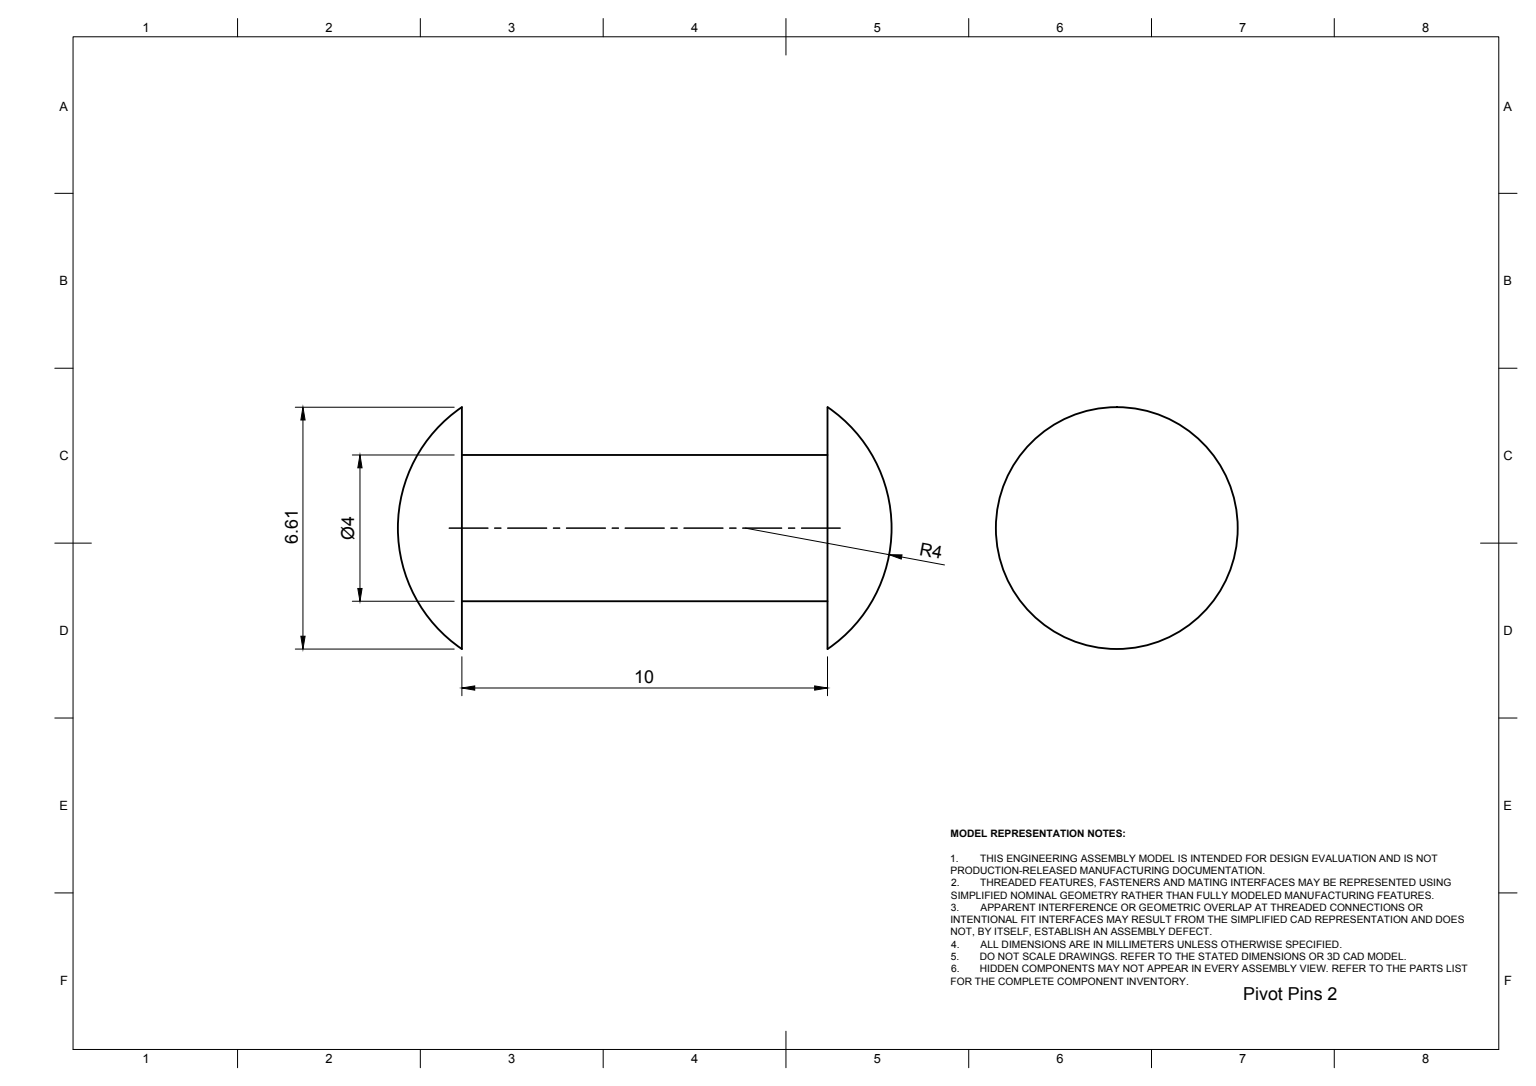
ISO-10303-21;
HEADER;
/* Generated by software containing ST-Developer
 * from STEP Tools, Inc. (www.steptools.com) 
 */

FILE_DESCRIPTION(
/* description */ ('STEP AP214'),
/* implementation_level */ '2;1');

FILE_NAME(
/* name */ 'Pivot Pins 2.step',
/* time_stamp */ '2026-10-06T11:11:25-07:00',
/* author */ (''),
/* organization */ (''),
/* preprocessor_version */ 'ST-DEVELOPER v20.2',
/* originating_system */ 'Autodesk Translation Framework v15.15.0.0',
/* authorisation */ '');

FILE_SCHEMA (('AUTOMOTIVE_DESIGN { 1 0 10303 214 3 1 1 }'));
ENDSEC;

DATA;
#10=MECHANICAL_DESIGN_GEOMETRIC_PRESENTATION_REPRESENTATION('',(#707),#47717);
#683=SHAPE_REPRESENTATION_RELATIONSHIP('SRR','None',#47770,#695);
#695=ADVANCED_BREP_SHAPE_REPRESENTATION('',(#719),#47714);
#707=STYLED_ITEM('',(#47830),#719);
#719=MANIFOLD_SOLID_BREP('Body1',#8934);
#751=FACE_BOUND('',#3058,.T.);
#752=FACE_BOUND('',#3060,.T.);
#871=PLANE('',#9832);
#872=PLANE('',#9833);
#1330=LINE('',#45925,#1817);
#1817=VECTOR('',#11921,2.);
#2041=CYLINDRICAL_SURFACE('',#9827,2.);
#2513=FACE_OUTER_BOUND('',#3054,.T.);
#2514=FACE_OUTER_BOUND('',#3055,.T.);
#2515=FACE_OUTER_BOUND('',#3056,.T.);
#2516=FACE_OUTER_BOUND('',#3057,.T.);
#2517=FACE_OUTER_BOUND('',#3059,.T.);
#3054=EDGE_LOOP('',(#8115));
#3055=EDGE_LOOP('',(#8116,#8117,#8118,#8119));
#3056=EDGE_LOOP('',(#8120));
#3057=EDGE_LOOP('',(#8121));
#3058=EDGE_LOOP('',(#8122));
#3059=EDGE_LOOP('',(#8123));
#3060=EDGE_LOOP('',(#8124));
#3468=CIRCLE('',#9826,3.30718913883074);
#3469=CIRCLE('',#9828,2.);
#3470=CIRCLE('',#9829,2.);
#3471=CIRCLE('',#9831,3.30718913883074);
#4301=VERTEX_POINT('',#45919);
#4302=VERTEX_POINT('',#45922);
#4303=VERTEX_POINT('',#45924);
#4304=VERTEX_POINT('',#45928);
#5583=EDGE_CURVE('',#4301,#4301,#3468,.T.);
#5584=EDGE_CURVE('',#4302,#4302,#3469,.T.);
#5585=EDGE_CURVE('',#4302,#4303,#1330,.T.);
#5586=EDGE_CURVE('',#4303,#4303,#3470,.T.);
#5587=EDGE_CURVE('',#4304,#4304,#3471,.T.);
#8115=ORIENTED_EDGE('',*,*,#5583,.T.);
#8116=ORIENTED_EDGE('',*,*,#5584,.F.);
#8117=ORIENTED_EDGE('',*,*,#5585,.T.);
#8118=ORIENTED_EDGE('',*,*,#5586,.T.);
#8119=ORIENTED_EDGE('',*,*,#5585,.F.);
#8120=ORIENTED_EDGE('',*,*,#5587,.F.);
#8121=ORIENTED_EDGE('',*,*,#5587,.T.);
#8122=ORIENTED_EDGE('',*,*,#5586,.F.);
#8123=ORIENTED_EDGE('',*,*,#5583,.F.);
#8124=ORIENTED_EDGE('',*,*,#5584,.T.);
#8411=SPHERICAL_SURFACE('',#9825,4.);
#8412=SPHERICAL_SURFACE('',#9830,4.);
#8863=ADVANCED_FACE('',(#2513),#8411,.T.);
#8864=ADVANCED_FACE('',(#2514),#2041,.T.);
#8865=ADVANCED_FACE('',(#2515),#8412,.T.);
#8866=ADVANCED_FACE('',(#2516,#751),#871,.T.);
#8867=ADVANCED_FACE('',(#2517,#752),#872,.T.);
#8934=CLOSED_SHELL('',(#8863,#8864,#8865,#8866,#8867));
#9824=AXIS2_PLACEMENT_3D('',#45917,#11911,#11912);
#9825=AXIS2_PLACEMENT_3D('',#45918,#11913,#11914);
#9826=AXIS2_PLACEMENT_3D('',#45920,#11915,#11916);
#9827=AXIS2_PLACEMENT_3D('',#45921,#11917,#11918);
#9828=AXIS2_PLACEMENT_3D('',#45923,#11919,#11920);
#9829=AXIS2_PLACEMENT_3D('',#45926,#11922,#11923);
#9830=AXIS2_PLACEMENT_3D('',#45927,#11924,#11925);
#9831=AXIS2_PLACEMENT_3D('',#45929,#11926,#11927);
#9832=AXIS2_PLACEMENT_3D('',#45930,#11928,#11929);
#9833=AXIS2_PLACEMENT_3D('',#45931,#11930,#11931);
#11911=DIRECTION('axis',(0.,0.,1.));
#11912=DIRECTION('refdir',(1.,0.,0.));
#11913=DIRECTION('center_axis',(0.00483401456277122,-0.999988316083346,
0.));
#11914=DIRECTION('ref_axis',(0.999988316083346,0.00483401456277122,0.));
#11915=DIRECTION('center_axis',(2.50063434304146E-17,1.27632226958495E-16,
1.));
#11916=DIRECTION('ref_axis',(0.00483401456277147,-0.999988316083347,1.27509854685889E-16));
#11917=DIRECTION('center_axis',(2.50063434304146E-17,1.27632226958495E-16,
1.));
#11918=DIRECTION('ref_axis',(0.00483401456276983,-0.999988316083346,1.27509854685889E-16));
#11919=DIRECTION('center_axis',(2.50063434304146E-17,1.27632226958495E-16,
1.));
#11920=DIRECTION('ref_axis',(0.00483401456276983,-0.999988316083346,1.27509854685889E-16));
#11921=DIRECTION('',(-2.50063434304146E-17,-1.27632226958495E-16,-1.));
#11922=DIRECTION('center_axis',(2.50063434304146E-17,1.27632226958495E-16,
1.));
#11923=DIRECTION('ref_axis',(0.00483401456276983,-0.999988316083346,1.27509854685889E-16));
#11924=DIRECTION('center_axis',(-0.00483401456277122,0.999988316083346,
0.));
#11925=DIRECTION('ref_axis',(0.999988316083346,0.00483401456277122,0.));
#11926=DIRECTION('center_axis',(2.50063434304146E-17,1.27632226958495E-16,
1.));
#11927=DIRECTION('ref_axis',(0.00483401456277147,-0.999988316083347,1.27509854685889E-16));
#11928=DIRECTION('center_axis',(2.50063434304146E-17,1.27632226958495E-16,
1.));
#11929=DIRECTION('ref_axis',(0.00483401456277099,-0.999988316083347,1.27509854685889E-16));
#11930=DIRECTION('center_axis',(-2.50063434304146E-17,-1.27632226958495E-16,
-1.));
#11931=DIRECTION('ref_axis',(0.00483401456277099,-0.999988316083347,1.27509854685889E-16));
#45917=CARTESIAN_POINT('',(0.,0.,0.));
#45918=CARTESIAN_POINT('Origin',(-70.1438101352769,-11.0431453779948,178.735485069079));
#45919=CARTESIAN_POINT('',(-73.4509606331853,-11.0591323784537,180.985485069079));
#45920=CARTESIAN_POINT('Origin',(-70.1438101352769,-11.0431453779948,180.985485069079));
#45921=CARTESIAN_POINT('Origin',(-70.1438101352769,-11.0431453779948,175.985485069079));
#45922=CARTESIAN_POINT('',(-70.1534781644024,-9.04316874582809,180.985485069079));
#45923=CARTESIAN_POINT('Origin',(-70.1438101352769,-11.0431453779948,180.985485069079));
#45924=CARTESIAN_POINT('',(-70.1534781644024,-9.04316874582809,170.985485069079));
#45925=CARTESIAN_POINT('',(-70.1534781644024,-9.04316874582809,175.985485069079));
#45926=CARTESIAN_POINT('Origin',(-70.1438101352769,-11.0431453779948,170.985485069079));
#45927=CARTESIAN_POINT('Origin',(-70.1438101352769,-11.0431453779948,173.235485069079));
#45928=CARTESIAN_POINT('',(-73.4509606331853,-11.0591323784537,170.985485069079));
#45929=CARTESIAN_POINT('Origin',(-70.1438101352769,-11.0431453779948,170.985485069079));
#45930=CARTESIAN_POINT('Origin',(-68.1438335031102,-11.0334773488692,170.985485069079));
#45931=CARTESIAN_POINT('Origin',(-68.1438335031102,-11.0334773488692,180.985485069079));
#47700=UNCERTAINTY_MEASURE_WITH_UNIT(LENGTH_MEASURE(0.01),#47718,
'DISTANCE_ACCURACY_VALUE',
'Maximum model space distance between geometric entities at asserted c
onnectivities');
#47703=UNCERTAINTY_MEASURE_WITH_UNIT(LENGTH_MEASURE(0.01),#47718,
'DISTANCE_ACCURACY_VALUE',
'Maximum model space distance between geometric entities at asserted c
onnectivities');
#47714=(
GEOMETRIC_REPRESENTATION_CONTEXT(3)
GLOBAL_UNCERTAINTY_ASSIGNED_CONTEXT((#47700))
GLOBAL_UNIT_ASSIGNED_CONTEXT((#47718,#47720,#47721))
REPRESENTATION_CONTEXT('','3D')
);
#47717=(
GEOMETRIC_REPRESENTATION_CONTEXT(3)
GLOBAL_UNCERTAINTY_ASSIGNED_CONTEXT((#47703))
GLOBAL_UNIT_ASSIGNED_CONTEXT((#47718,#47720,#47721))
REPRESENTATION_CONTEXT('','3D')
);
#47718=(
LENGTH_UNIT()
NAMED_UNIT(*)
SI_UNIT(.MILLI.,.METRE.)
);
#47720=(
NAMED_UNIT(*)
PLANE_ANGLE_UNIT()
SI_UNIT($,.RADIAN.)
);
#47721=(
NAMED_UNIT(*)
SI_UNIT($,.STERADIAN.)
SOLID_ANGLE_UNIT()
);
#47732=SHAPE_DEFINITION_REPRESENTATION(#47745,#47770);
#47745=PRODUCT_DEFINITION_SHAPE('',$,#47784);
#47770=SHAPE_REPRESENTATION('',(#9824),#47714);
#47773=PRODUCT_DEFINITION_CONTEXT('part definition',#47814,'design');
#47784=PRODUCT_DEFINITION('Pivot Pins 2','Pivot Pins 2',#47797,#47773);
#47797=PRODUCT_DEFINITION_FORMATION('',$,#47826);
#47814=APPLICATION_CONTEXT(
'Core Data for Automotive Mechanical Design Process');
#47815=PRODUCT_CONTEXT('part definition',#47814,'mechanical');
#47826=PRODUCT('Pivot Pins 2','Pivot Pins 2',$,(#47815));
#47830=PRESENTATION_STYLE_ASSIGNMENT((#47832));
#47832=SURFACE_STYLE_USAGE(.BOTH.,#47834);
#47834=SURFACE_SIDE_STYLE('',(#47836));
#47836=SURFACE_STYLE_FILL_AREA(#47838);
#47838=FILL_AREA_STYLE('Opaque(202,209,238)',(#47840));
#47840=FILL_AREA_STYLE_COLOUR('Opaque(202,209,238)',#47842);
#47842=COLOUR_RGB('Opaque(202,209,238)', 0.66274510, 0.83137255, 0.94901961);
ENDSEC;
END-ISO-10303-21;
